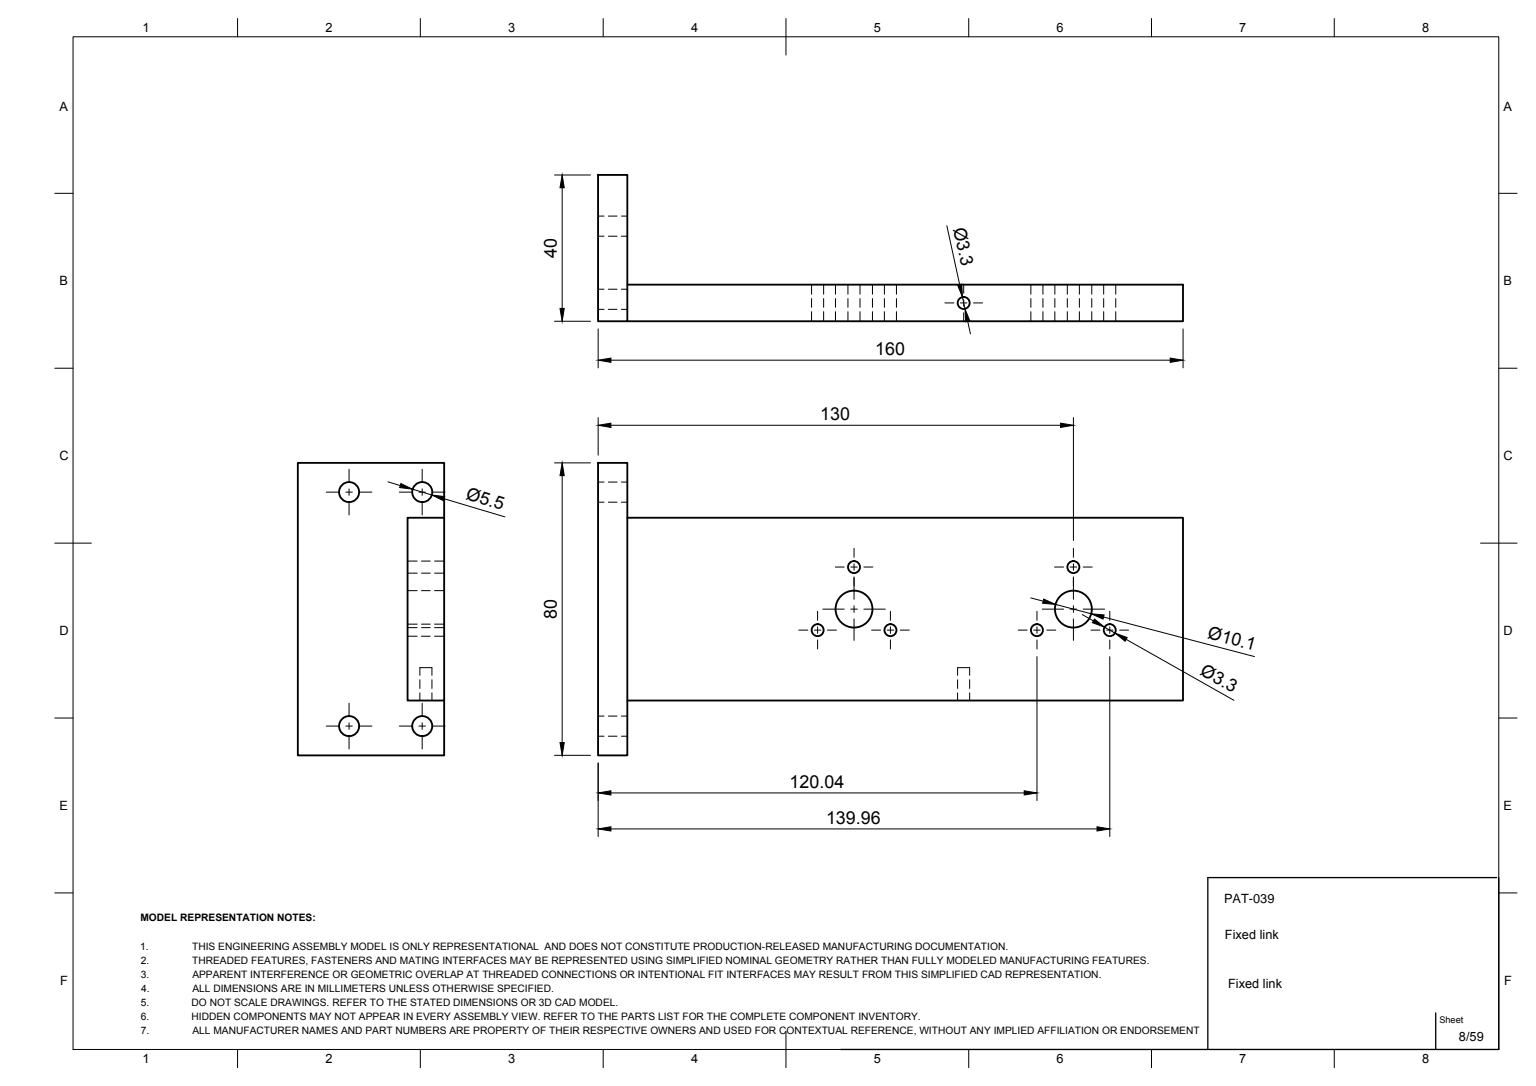
ISO-10303-21;
HEADER;
/* Generated by software containing ST-Developer
 * from STEP Tools, Inc. (www.steptools.com) 
 */

FILE_DESCRIPTION(
/* description */ ('Four-bar parallelogram arm'),
/* implementation_level */ '2;1');

FILE_NAME(
/* name */ 'Fixed link.step',
/* time_stamp */ '2026-10-28T03:24:55-07:00',
/* author */ (''),
/* organization */ (''),
/* preprocessor_version */ 'ST-DEVELOPER v20.2',
/* originating_system */ 'Autodesk Translation Framework v15.17.0.0',
/* authorisation */ '');

FILE_SCHEMA (('AUTOMOTIVE_DESIGN { 1 0 10303 214 3 1 1 }'));
ENDSEC;

DATA;
#10=MECHANICAL_DESIGN_GEOMETRIC_PRESENTATION_REPRESENTATION('',(#625),#14512);
#525=SHAPE_REPRESENTATION_RELATIONSHIP('SRR','None',#14746,#575);
#575=ADVANCED_BREP_SHAPE_REPRESENTATION('',(#683),#14461);
#625=STYLED_ITEM('',(#15101),#683);
#683=MANIFOLD_SOLID_BREP('Body1',#7329);
#743=FACE_BOUND('',#1666,.T.);
#744=FACE_BOUND('',#1667,.T.);
#745=FACE_BOUND('',#1668,.T.);
#746=FACE_BOUND('',#1669,.T.);
#747=FACE_BOUND('',#1672,.T.);
#748=FACE_BOUND('',#1673,.T.);
#749=FACE_BOUND('',#1674,.T.);
#750=FACE_BOUND('',#1675,.T.);
#751=FACE_BOUND('',#1679,.T.);
#752=FACE_BOUND('',#1680,.T.);
#753=FACE_BOUND('',#1681,.T.);
#754=FACE_BOUND('',#1682,.T.);
#755=FACE_BOUND('',#1683,.T.);
#756=FACE_BOUND('',#1684,.T.);
#757=FACE_BOUND('',#1685,.T.);
#758=FACE_BOUND('',#1686,.T.);
#759=FACE_BOUND('',#1689,.T.);
#760=FACE_BOUND('',#1690,.T.);
#761=FACE_BOUND('',#1691,.T.);
#762=FACE_BOUND('',#1692,.T.);
#763=FACE_BOUND('',#1693,.T.);
#764=FACE_BOUND('',#1694,.T.);
#765=FACE_BOUND('',#1695,.T.);
#766=FACE_BOUND('',#1696,.T.);
#767=FACE_BOUND('',#1698,.T.);
#1024=PLANE('',#7977);
#1025=PLANE('',#8014);
#1026=PLANE('',#8015);
#1027=PLANE('',#8016);
#1028=PLANE('',#8017);
#1029=PLANE('',#8018);
#1030=PLANE('',#8019);
#1031=PLANE('',#8020);
#1032=PLANE('',#8021);
#1033=PLANE('',#8022);
#1034=PLANE('',#8023);
#1223=FACE_OUTER_BOUND('',#1651,.T.);
#1224=FACE_OUTER_BOUND('',#1652,.T.);
#1225=FACE_OUTER_BOUND('',#1653,.T.);
#1226=FACE_OUTER_BOUND('',#1654,.T.);
#1227=FACE_OUTER_BOUND('',#1655,.T.);
#1228=FACE_OUTER_BOUND('',#1656,.T.);
#1229=FACE_OUTER_BOUND('',#1657,.T.);
#1230=FACE_OUTER_BOUND('',#1658,.T.);
#1231=FACE_OUTER_BOUND('',#1659,.T.);
#1232=FACE_OUTER_BOUND('',#1660,.T.);
#1233=FACE_OUTER_BOUND('',#1661,.T.);
#1234=FACE_OUTER_BOUND('',#1662,.T.);
#1235=FACE_OUTER_BOUND('',#1663,.T.);
#1236=FACE_OUTER_BOUND('',#1664,.T.);
#1237=FACE_OUTER_BOUND('',#1665,.T.);
#1238=FACE_OUTER_BOUND('',#1670,.T.);
#1239=FACE_OUTER_BOUND('',#1671,.T.);
#1240=FACE_OUTER_BOUND('',#1676,.T.);
#1241=FACE_OUTER_BOUND('',#1677,.T.);
#1242=FACE_OUTER_BOUND('',#1678,.T.);
#1243=FACE_OUTER_BOUND('',#1687,.T.);
#1244=FACE_OUTER_BOUND('',#1688,.T.);
#1245=FACE_OUTER_BOUND('',#1697,.T.);
#1246=FACE_OUTER_BOUND('',#1699,.T.);
#1651=EDGE_LOOP('',(#5084,#5085,#5086,#5087));
#1652=EDGE_LOOP('',(#5088));
#1653=EDGE_LOOP('',(#5089,#5090,#5091,#5092));
#1654=EDGE_LOOP('',(#5093,#5094,#5095,#5096));
#1655=EDGE_LOOP('',(#5097,#5098,#5099,#5100));
#1656=EDGE_LOOP('',(#5101,#5102,#5103,#5104));
#1657=EDGE_LOOP('',(#5105,#5106,#5107,#5108));
#1658=EDGE_LOOP('',(#5109,#5110,#5111,#5112));
#1659=EDGE_LOOP('',(#5113,#5114,#5115,#5116));
#1660=EDGE_LOOP('',(#5117,#5118,#5119,#5120));
#1661=EDGE_LOOP('',(#5121,#5122,#5123,#5124));
#1662=EDGE_LOOP('',(#5125,#5126,#5127,#5128));
#1663=EDGE_LOOP('',(#5129,#5130,#5131,#5132));
#1664=EDGE_LOOP('',(#5133,#5134,#5135,#5136));
#1665=EDGE_LOOP('',(#5137,#5138,#5139,#5140,#5141,#5142,#5143,#5144));
#1666=EDGE_LOOP('',(#5145));
#1667=EDGE_LOOP('',(#5146));
#1668=EDGE_LOOP('',(#5147));
#1669=EDGE_LOOP('',(#5148));
#1670=EDGE_LOOP('',(#5149,#5150,#5151,#5152));
#1671=EDGE_LOOP('',(#5153,#5154,#5155,#5156));
#1672=EDGE_LOOP('',(#5157));
#1673=EDGE_LOOP('',(#5158));
#1674=EDGE_LOOP('',(#5159));
#1675=EDGE_LOOP('',(#5160));
#1676=EDGE_LOOP('',(#5161,#5162,#5163,#5164));
#1677=EDGE_LOOP('',(#5165,#5166,#5167,#5168));
#1678=EDGE_LOOP('',(#5169,#5170,#5171,#5172));
#1679=EDGE_LOOP('',(#5173));
#1680=EDGE_LOOP('',(#5174));
#1681=EDGE_LOOP('',(#5175));
#1682=EDGE_LOOP('',(#5176));
#1683=EDGE_LOOP('',(#5177));
#1684=EDGE_LOOP('',(#5178));
#1685=EDGE_LOOP('',(#5179));
#1686=EDGE_LOOP('',(#5180));
#1687=EDGE_LOOP('',(#5181,#5182,#5183,#5184));
#1688=EDGE_LOOP('',(#5185,#5186,#5187,#5188,#5189,#5190,#5191,#5192));
#1689=EDGE_LOOP('',(#5193));
#1690=EDGE_LOOP('',(#5194));
#1691=EDGE_LOOP('',(#5195));
#1692=EDGE_LOOP('',(#5196));
#1693=EDGE_LOOP('',(#5197));
#1694=EDGE_LOOP('',(#5198));
#1695=EDGE_LOOP('',(#5199));
#1696=EDGE_LOOP('',(#5200));
#1697=EDGE_LOOP('',(#5201,#5202,#5203,#5204));
#1698=EDGE_LOOP('',(#5205));
#1699=EDGE_LOOP('',(#5206,#5207,#5208,#5209));
#2352=LINE('',#11540,#2746);
#2353=LINE('',#11547,#2747);
#2354=LINE('',#11553,#2748);
#2355=LINE('',#11559,#2749);
#2356=LINE('',#11565,#2750);
#2357=LINE('',#11571,#2751);
#2358=LINE('',#11577,#2752);
#2359=LINE('',#11583,#2753);
#2360=LINE('',#11589,#2754);
#2361=LINE('',#11595,#2755);
#2362=LINE('',#11601,#2756);
#2363=LINE('',#11607,#2757);
#2364=LINE('',#11613,#2758);
#2365=LINE('',#11618,#2759);
#2366=LINE('',#11620,#2760);
#2367=LINE('',#11622,#2761);
#2368=LINE('',#11624,#2762);
#2369=LINE('',#11626,#2763);
#2370=LINE('',#11628,#2764);
#2371=LINE('',#11630,#2765);
#2372=LINE('',#11631,#2766);
#2373=LINE('',#11634,#2767);
#2374=LINE('',#11636,#2768);
#2375=LINE('',#11637,#2769);
#2376=LINE('',#11640,#2770);
#2377=LINE('',#11642,#2771);
#2378=LINE('',#11643,#2772);
#2379=LINE('',#11645,#2773);
#2380=LINE('',#11646,#2774);
#2381=LINE('',#11650,#2775);
#2382=LINE('',#11652,#2776);
#2383=LINE('',#11653,#2777);
#2384=LINE('',#11656,#2778);
#2385=LINE('',#11657,#2779);
#2386=LINE('',#11660,#2780);
#2387=LINE('',#11661,#2781);
#2388=LINE('',#11663,#2782);
#2746=VECTOR('',#9086,0.164999999999999);
#2747=VECTOR('',#9095,0.165);
#2748=VECTOR('',#9102,0.165);
#2749=VECTOR('',#9109,0.165);
#2750=VECTOR('',#9116,0.505);
#2751=VECTOR('',#9123,0.165);
#2752=VECTOR('',#9130,0.165);
#2753=VECTOR('',#9137,0.165);
#2754=VECTOR('',#9144,0.505);
#2755=VECTOR('',#9151,0.275);
#2756=VECTOR('',#9158,0.275);
#2757=VECTOR('',#9165,0.275);
#2758=VECTOR('',#9172,0.275);
#2759=VECTOR('',#9177,1.);
#2760=VECTOR('',#9178,1.);
#2761=VECTOR('',#9179,1.);
#2762=VECTOR('',#9180,1.);
#2763=VECTOR('',#9181,1.);
#2764=VECTOR('',#9182,1.);
#2765=VECTOR('',#9183,1.);
#2766=VECTOR('',#9184,1.);
#2767=VECTOR('',#9187,1.);
#2768=VECTOR('',#9188,1.);
#2769=VECTOR('',#9189,1.);
#2770=VECTOR('',#9192,1.);
#2771=VECTOR('',#9193,1.);
#2772=VECTOR('',#9194,1.);
#2773=VECTOR('',#9197,1.);
#2774=VECTOR('',#9198,1.);
#2775=VECTOR('',#9203,1.);
#2776=VECTOR('',#9204,1.);
#2777=VECTOR('',#9205,1.);
#2778=VECTOR('',#9208,1.);
#2779=VECTOR('',#9209,1.);
#2780=VECTOR('',#9212,1.);
#2781=VECTOR('',#9213,1.);
#2782=VECTOR('',#9216,1.);
#3108=CIRCLE('',#7975,0.164999999999999);
#3109=CIRCLE('',#7976,0.164999999999999);
#3110=CIRCLE('',#7979,0.165);
#3111=CIRCLE('',#7980,0.165);
#3112=CIRCLE('',#7982,0.165);
#3113=CIRCLE('',#7983,0.165);
#3114=CIRCLE('',#7985,0.165);
#3115=CIRCLE('',#7986,0.165);
#3116=CIRCLE('',#7988,0.505);
#3117=CIRCLE('',#7989,0.505);
#3118=CIRCLE('',#7991,0.165);
#3119=CIRCLE('',#7992,0.165);
#3120=CIRCLE('',#7994,0.165);
#3121=CIRCLE('',#7995,0.165);
#3122=CIRCLE('',#7997,0.165);
#3123=CIRCLE('',#7998,0.165);
#3124=CIRCLE('',#8000,0.505);
#3125=CIRCLE('',#8001,0.505);
#3126=CIRCLE('',#8003,0.275);
#3127=CIRCLE('',#8004,0.275);
#3128=CIRCLE('',#8006,0.275);
#3129=CIRCLE('',#8007,0.275);
#3130=CIRCLE('',#8009,0.275);
#3131=CIRCLE('',#8010,0.275);
#3132=CIRCLE('',#8012,0.275);
#3133=CIRCLE('',#8013,0.275);
#3577=VERTEX_POINT('',#11537);
#3578=VERTEX_POINT('',#11539);
#3579=VERTEX_POINT('',#11544);
#3580=VERTEX_POINT('',#11546);
#3581=VERTEX_POINT('',#11550);
#3582=VERTEX_POINT('',#11552);
#3583=VERTEX_POINT('',#11556);
#3584=VERTEX_POINT('',#11558);
#3585=VERTEX_POINT('',#11562);
#3586=VERTEX_POINT('',#11564);
#3587=VERTEX_POINT('',#11568);
#3588=VERTEX_POINT('',#11570);
#3589=VERTEX_POINT('',#11574);
#3590=VERTEX_POINT('',#11576);
#3591=VERTEX_POINT('',#11580);
#3592=VERTEX_POINT('',#11582);
#3593=VERTEX_POINT('',#11586);
#3594=VERTEX_POINT('',#11588);
#3595=VERTEX_POINT('',#11592);
#3596=VERTEX_POINT('',#11594);
#3597=VERTEX_POINT('',#11598);
#3598=VERTEX_POINT('',#11600);
#3599=VERTEX_POINT('',#11604);
#3600=VERTEX_POINT('',#11606);
#3601=VERTEX_POINT('',#11610);
#3602=VERTEX_POINT('',#11612);
#3603=VERTEX_POINT('',#11616);
#3604=VERTEX_POINT('',#11617);
#3605=VERTEX_POINT('',#11619);
#3606=VERTEX_POINT('',#11621);
#3607=VERTEX_POINT('',#11623);
#3608=VERTEX_POINT('',#11625);
#3609=VERTEX_POINT('',#11627);
#3610=VERTEX_POINT('',#11629);
#3611=VERTEX_POINT('',#11633);
#3612=VERTEX_POINT('',#11635);
#3613=VERTEX_POINT('',#11639);
#3614=VERTEX_POINT('',#11641);
#3615=VERTEX_POINT('',#11649);
#3616=VERTEX_POINT('',#11651);
#3617=VERTEX_POINT('',#11655);
#3618=VERTEX_POINT('',#11659);
#4173=EDGE_CURVE('',#3577,#3577,#3108,.T.);
#4174=EDGE_CURVE('',#3577,#3578,#2352,.T.);
#4175=EDGE_CURVE('',#3578,#3578,#3109,.T.);
#4176=EDGE_CURVE('',#3579,#3579,#3110,.T.);
#4177=EDGE_CURVE('',#3579,#3580,#2353,.T.);
#4178=EDGE_CURVE('',#3580,#3580,#3111,.T.);
#4179=EDGE_CURVE('',#3581,#3581,#3112,.T.);
#4180=EDGE_CURVE('',#3581,#3582,#2354,.T.);
#4181=EDGE_CURVE('',#3582,#3582,#3113,.T.);
#4182=EDGE_CURVE('',#3583,#3583,#3114,.T.);
#4183=EDGE_CURVE('',#3583,#3584,#2355,.T.);
#4184=EDGE_CURVE('',#3584,#3584,#3115,.T.);
#4185=EDGE_CURVE('',#3585,#3585,#3116,.T.);
#4186=EDGE_CURVE('',#3585,#3586,#2356,.T.);
#4187=EDGE_CURVE('',#3586,#3586,#3117,.T.);
#4188=EDGE_CURVE('',#3587,#3587,#3118,.T.);
#4189=EDGE_CURVE('',#3587,#3588,#2357,.T.);
#4190=EDGE_CURVE('',#3588,#3588,#3119,.T.);
#4191=EDGE_CURVE('',#3589,#3589,#3120,.T.);
#4192=EDGE_CURVE('',#3589,#3590,#2358,.T.);
#4193=EDGE_CURVE('',#3590,#3590,#3121,.T.);
#4194=EDGE_CURVE('',#3591,#3591,#3122,.T.);
#4195=EDGE_CURVE('',#3591,#3592,#2359,.T.);
#4196=EDGE_CURVE('',#3592,#3592,#3123,.T.);
#4197=EDGE_CURVE('',#3593,#3593,#3124,.T.);
#4198=EDGE_CURVE('',#3593,#3594,#2360,.T.);
#4199=EDGE_CURVE('',#3594,#3594,#3125,.T.);
#4200=EDGE_CURVE('',#3595,#3595,#3126,.T.);
#4201=EDGE_CURVE('',#3595,#3596,#2361,.T.);
#4202=EDGE_CURVE('',#3596,#3596,#3127,.T.);
#4203=EDGE_CURVE('',#3597,#3597,#3128,.T.);
#4204=EDGE_CURVE('',#3597,#3598,#2362,.T.);
#4205=EDGE_CURVE('',#3598,#3598,#3129,.T.);
#4206=EDGE_CURVE('',#3599,#3599,#3130,.T.);
#4207=EDGE_CURVE('',#3599,#3600,#2363,.T.);
#4208=EDGE_CURVE('',#3600,#3600,#3131,.T.);
#4209=EDGE_CURVE('',#3601,#3601,#3132,.T.);
#4210=EDGE_CURVE('',#3601,#3602,#2364,.T.);
#4211=EDGE_CURVE('',#3602,#3602,#3133,.T.);
#4212=EDGE_CURVE('',#3603,#3604,#2365,.T.);
#4213=EDGE_CURVE('',#3605,#3603,#2366,.T.);
#4214=EDGE_CURVE('',#3606,#3605,#2367,.T.);
#4215=EDGE_CURVE('',#3607,#3606,#2368,.T.);
#4216=EDGE_CURVE('',#3607,#3608,#2369,.T.);
#4217=EDGE_CURVE('',#3609,#3608,#2370,.T.);
#4218=EDGE_CURVE('',#3610,#3609,#2371,.T.);
#4219=EDGE_CURVE('',#3604,#3610,#2372,.T.);
#4220=EDGE_CURVE('',#3610,#3611,#2373,.T.);
#4221=EDGE_CURVE('',#3612,#3609,#2374,.T.);
#4222=EDGE_CURVE('',#3611,#3612,#2375,.T.);
#4223=EDGE_CURVE('',#3611,#3613,#2376,.T.);
#4224=EDGE_CURVE('',#3614,#3612,#2377,.T.);
#4225=EDGE_CURVE('',#3613,#3614,#2378,.T.);
#4226=EDGE_CURVE('',#3613,#3607,#2379,.T.);
#4227=EDGE_CURVE('',#3608,#3614,#2380,.T.);
#4228=EDGE_CURVE('',#3603,#3615,#2381,.T.);
#4229=EDGE_CURVE('',#3616,#3615,#2382,.T.);
#4230=EDGE_CURVE('',#3605,#3616,#2383,.T.);
#4231=EDGE_CURVE('',#3617,#3616,#2384,.T.);
#4232=EDGE_CURVE('',#3606,#3617,#2385,.T.);
#4233=EDGE_CURVE('',#3618,#3617,#2386,.T.);
#4234=EDGE_CURVE('',#3604,#3618,#2387,.T.);
#4235=EDGE_CURVE('',#3615,#3618,#2388,.T.);
#5084=ORIENTED_EDGE('',*,*,#4173,.F.);
#5085=ORIENTED_EDGE('',*,*,#4174,.T.);
#5086=ORIENTED_EDGE('',*,*,#4175,.T.);
#5087=ORIENTED_EDGE('',*,*,#4174,.F.);
#5088=ORIENTED_EDGE('',*,*,#4175,.F.);
#5089=ORIENTED_EDGE('',*,*,#4176,.F.);
#5090=ORIENTED_EDGE('',*,*,#4177,.T.);
#5091=ORIENTED_EDGE('',*,*,#4178,.F.);
#5092=ORIENTED_EDGE('',*,*,#4177,.F.);
#5093=ORIENTED_EDGE('',*,*,#4179,.F.);
#5094=ORIENTED_EDGE('',*,*,#4180,.T.);
#5095=ORIENTED_EDGE('',*,*,#4181,.F.);
#5096=ORIENTED_EDGE('',*,*,#4180,.F.);
#5097=ORIENTED_EDGE('',*,*,#4182,.F.);
#5098=ORIENTED_EDGE('',*,*,#4183,.T.);
#5099=ORIENTED_EDGE('',*,*,#4184,.F.);
#5100=ORIENTED_EDGE('',*,*,#4183,.F.);
#5101=ORIENTED_EDGE('',*,*,#4185,.F.);
#5102=ORIENTED_EDGE('',*,*,#4186,.T.);
#5103=ORIENTED_EDGE('',*,*,#4187,.F.);
#5104=ORIENTED_EDGE('',*,*,#4186,.F.);
#5105=ORIENTED_EDGE('',*,*,#4188,.F.);
#5106=ORIENTED_EDGE('',*,*,#4189,.T.);
#5107=ORIENTED_EDGE('',*,*,#4190,.F.);
#5108=ORIENTED_EDGE('',*,*,#4189,.F.);
#5109=ORIENTED_EDGE('',*,*,#4191,.F.);
#5110=ORIENTED_EDGE('',*,*,#4192,.T.);
#5111=ORIENTED_EDGE('',*,*,#4193,.F.);
#5112=ORIENTED_EDGE('',*,*,#4192,.F.);
#5113=ORIENTED_EDGE('',*,*,#4194,.F.);
#5114=ORIENTED_EDGE('',*,*,#4195,.T.);
#5115=ORIENTED_EDGE('',*,*,#4196,.F.);
#5116=ORIENTED_EDGE('',*,*,#4195,.F.);
#5117=ORIENTED_EDGE('',*,*,#4197,.F.);
#5118=ORIENTED_EDGE('',*,*,#4198,.T.);
#5119=ORIENTED_EDGE('',*,*,#4199,.F.);
#5120=ORIENTED_EDGE('',*,*,#4198,.F.);
#5121=ORIENTED_EDGE('',*,*,#4200,.F.);
#5122=ORIENTED_EDGE('',*,*,#4201,.T.);
#5123=ORIENTED_EDGE('',*,*,#4202,.F.);
#5124=ORIENTED_EDGE('',*,*,#4201,.F.);
#5125=ORIENTED_EDGE('',*,*,#4203,.F.);
#5126=ORIENTED_EDGE('',*,*,#4204,.T.);
#5127=ORIENTED_EDGE('',*,*,#4205,.F.);
#5128=ORIENTED_EDGE('',*,*,#4204,.F.);
#5129=ORIENTED_EDGE('',*,*,#4206,.F.);
#5130=ORIENTED_EDGE('',*,*,#4207,.T.);
#5131=ORIENTED_EDGE('',*,*,#4208,.F.);
#5132=ORIENTED_EDGE('',*,*,#4207,.F.);
#5133=ORIENTED_EDGE('',*,*,#4209,.F.);
#5134=ORIENTED_EDGE('',*,*,#4210,.T.);
#5135=ORIENTED_EDGE('',*,*,#4211,.F.);
#5136=ORIENTED_EDGE('',*,*,#4210,.F.);
#5137=ORIENTED_EDGE('',*,*,#4212,.F.);
#5138=ORIENTED_EDGE('',*,*,#4213,.F.);
#5139=ORIENTED_EDGE('',*,*,#4214,.F.);
#5140=ORIENTED_EDGE('',*,*,#4215,.F.);
#5141=ORIENTED_EDGE('',*,*,#4216,.T.);
#5142=ORIENTED_EDGE('',*,*,#4217,.F.);
#5143=ORIENTED_EDGE('',*,*,#4218,.F.);
#5144=ORIENTED_EDGE('',*,*,#4219,.F.);
#5145=ORIENTED_EDGE('',*,*,#4202,.T.);
#5146=ORIENTED_EDGE('',*,*,#4205,.T.);
#5147=ORIENTED_EDGE('',*,*,#4208,.T.);
#5148=ORIENTED_EDGE('',*,*,#4211,.T.);
#5149=ORIENTED_EDGE('',*,*,#4220,.F.);
#5150=ORIENTED_EDGE('',*,*,#4218,.T.);
#5151=ORIENTED_EDGE('',*,*,#4221,.F.);
#5152=ORIENTED_EDGE('',*,*,#4222,.F.);
#5153=ORIENTED_EDGE('',*,*,#4223,.F.);
#5154=ORIENTED_EDGE('',*,*,#4222,.T.);
#5155=ORIENTED_EDGE('',*,*,#4224,.F.);
#5156=ORIENTED_EDGE('',*,*,#4225,.F.);
#5157=ORIENTED_EDGE('',*,*,#4200,.T.);
#5158=ORIENTED_EDGE('',*,*,#4203,.T.);
#5159=ORIENTED_EDGE('',*,*,#4206,.T.);
#5160=ORIENTED_EDGE('',*,*,#4209,.T.);
#5161=ORIENTED_EDGE('',*,*,#4226,.F.);
#5162=ORIENTED_EDGE('',*,*,#4225,.T.);
#5163=ORIENTED_EDGE('',*,*,#4227,.F.);
#5164=ORIENTED_EDGE('',*,*,#4216,.F.);
#5165=ORIENTED_EDGE('',*,*,#4217,.T.);
#5166=ORIENTED_EDGE('',*,*,#4227,.T.);
#5167=ORIENTED_EDGE('',*,*,#4224,.T.);
#5168=ORIENTED_EDGE('',*,*,#4221,.T.);
#5169=ORIENTED_EDGE('',*,*,#4213,.T.);
#5170=ORIENTED_EDGE('',*,*,#4228,.T.);
#5171=ORIENTED_EDGE('',*,*,#4229,.F.);
#5172=ORIENTED_EDGE('',*,*,#4230,.F.);
#5173=ORIENTED_EDGE('',*,*,#4199,.T.);
#5174=ORIENTED_EDGE('',*,*,#4196,.T.);
#5175=ORIENTED_EDGE('',*,*,#4193,.T.);
#5176=ORIENTED_EDGE('',*,*,#4190,.T.);
#5177=ORIENTED_EDGE('',*,*,#4187,.T.);
#5178=ORIENTED_EDGE('',*,*,#4184,.T.);
#5179=ORIENTED_EDGE('',*,*,#4181,.T.);
#5180=ORIENTED_EDGE('',*,*,#4178,.T.);
#5181=ORIENTED_EDGE('',*,*,#4214,.T.);
#5182=ORIENTED_EDGE('',*,*,#4230,.T.);
#5183=ORIENTED_EDGE('',*,*,#4231,.F.);
#5184=ORIENTED_EDGE('',*,*,#4232,.F.);
#5185=ORIENTED_EDGE('',*,*,#4232,.T.);
#5186=ORIENTED_EDGE('',*,*,#4233,.F.);
#5187=ORIENTED_EDGE('',*,*,#4234,.F.);
#5188=ORIENTED_EDGE('',*,*,#4219,.T.);
#5189=ORIENTED_EDGE('',*,*,#4220,.T.);
#5190=ORIENTED_EDGE('',*,*,#4223,.T.);
#5191=ORIENTED_EDGE('',*,*,#4226,.T.);
#5192=ORIENTED_EDGE('',*,*,#4215,.T.);
#5193=ORIENTED_EDGE('',*,*,#4197,.T.);
#5194=ORIENTED_EDGE('',*,*,#4194,.T.);
#5195=ORIENTED_EDGE('',*,*,#4191,.T.);
#5196=ORIENTED_EDGE('',*,*,#4188,.T.);
#5197=ORIENTED_EDGE('',*,*,#4185,.T.);
#5198=ORIENTED_EDGE('',*,*,#4182,.T.);
#5199=ORIENTED_EDGE('',*,*,#4179,.T.);
#5200=ORIENTED_EDGE('',*,*,#4176,.T.);
#5201=ORIENTED_EDGE('',*,*,#4212,.T.);
#5202=ORIENTED_EDGE('',*,*,#4234,.T.);
#5203=ORIENTED_EDGE('',*,*,#4235,.F.);
#5204=ORIENTED_EDGE('',*,*,#4228,.F.);
#5205=ORIENTED_EDGE('',*,*,#4173,.T.);
#5206=ORIENTED_EDGE('',*,*,#4235,.T.);
#5207=ORIENTED_EDGE('',*,*,#4233,.T.);
#5208=ORIENTED_EDGE('',*,*,#4231,.T.);
#5209=ORIENTED_EDGE('',*,*,#4229,.T.);
#6718=CYLINDRICAL_SURFACE('',#7974,0.164999999999999);
#6719=CYLINDRICAL_SURFACE('',#7978,0.165);
#6720=CYLINDRICAL_SURFACE('',#7981,0.165);
#6721=CYLINDRICAL_SURFACE('',#7984,0.165);
#6722=CYLINDRICAL_SURFACE('',#7987,0.505);
#6723=CYLINDRICAL_SURFACE('',#7990,0.165);
#6724=CYLINDRICAL_SURFACE('',#7993,0.165);
#6725=CYLINDRICAL_SURFACE('',#7996,0.165);
#6726=CYLINDRICAL_SURFACE('',#7999,0.505);
#6727=CYLINDRICAL_SURFACE('',#8002,0.275);
#6728=CYLINDRICAL_SURFACE('',#8005,0.275);
#6729=CYLINDRICAL_SURFACE('',#8008,0.275);
#6730=CYLINDRICAL_SURFACE('',#8011,0.275);
#6928=ADVANCED_FACE('',(#1223),#6718,.F.);
#6929=ADVANCED_FACE('',(#1224),#1024,.F.);
#6930=ADVANCED_FACE('',(#1225),#6719,.F.);
#6931=ADVANCED_FACE('',(#1226),#6720,.F.);
#6932=ADVANCED_FACE('',(#1227),#6721,.F.);
#6933=ADVANCED_FACE('',(#1228),#6722,.F.);
#6934=ADVANCED_FACE('',(#1229),#6723,.F.);
#6935=ADVANCED_FACE('',(#1230),#6724,.F.);
#6936=ADVANCED_FACE('',(#1231),#6725,.F.);
#6937=ADVANCED_FACE('',(#1232),#6726,.F.);
#6938=ADVANCED_FACE('',(#1233),#6727,.F.);
#6939=ADVANCED_FACE('',(#1234),#6728,.F.);
#6940=ADVANCED_FACE('',(#1235),#6729,.F.);
#6941=ADVANCED_FACE('',(#1236),#6730,.F.);
#6942=ADVANCED_FACE('',(#1237,#743,#744,#745,#746),#1025,.T.);
#6943=ADVANCED_FACE('',(#1238),#1026,.T.);
#6944=ADVANCED_FACE('',(#1239,#747,#748,#749,#750),#1027,.T.);
#6945=ADVANCED_FACE('',(#1240),#1028,.T.);
#6946=ADVANCED_FACE('',(#1241),#1029,.T.);
#6947=ADVANCED_FACE('',(#1242,#751,#752,#753,#754,#755,#756,#757,#758),
#1030,.T.);
#6948=ADVANCED_FACE('',(#1243),#1031,.T.);
#6949=ADVANCED_FACE('',(#1244,#759,#760,#761,#762,#763,#764,#765,#766),
#1032,.T.);
#6950=ADVANCED_FACE('',(#1245,#767),#1033,.T.);
#6951=ADVANCED_FACE('',(#1246),#1034,.T.);
#7329=CLOSED_SHELL('',(#6928,#6929,#6930,#6931,#6932,#6933,#6934,#6935,
#6936,#6937,#6938,#6939,#6940,#6941,#6942,#6943,#6944,#6945,#6946,#6947,
#6948,#6949,#6950,#6951));
#7973=AXIS2_PLACEMENT_3D('',#11535,#9080,#9081);
#7974=AXIS2_PLACEMENT_3D('',#11536,#9082,#9083);
#7975=AXIS2_PLACEMENT_3D('',#11538,#9084,#9085);
#7976=AXIS2_PLACEMENT_3D('',#11541,#9087,#9088);
#7977=AXIS2_PLACEMENT_3D('',#11542,#9089,#9090);
#7978=AXIS2_PLACEMENT_3D('',#11543,#9091,#9092);
#7979=AXIS2_PLACEMENT_3D('',#11545,#9093,#9094);
#7980=AXIS2_PLACEMENT_3D('',#11548,#9096,#9097);
#7981=AXIS2_PLACEMENT_3D('',#11549,#9098,#9099);
#7982=AXIS2_PLACEMENT_3D('',#11551,#9100,#9101);
#7983=AXIS2_PLACEMENT_3D('',#11554,#9103,#9104);
#7984=AXIS2_PLACEMENT_3D('',#11555,#9105,#9106);
#7985=AXIS2_PLACEMENT_3D('',#11557,#9107,#9108);
#7986=AXIS2_PLACEMENT_3D('',#11560,#9110,#9111);
#7987=AXIS2_PLACEMENT_3D('',#11561,#9112,#9113);
#7988=AXIS2_PLACEMENT_3D('',#11563,#9114,#9115);
#7989=AXIS2_PLACEMENT_3D('',#11566,#9117,#9118);
#7990=AXIS2_PLACEMENT_3D('',#11567,#9119,#9120);
#7991=AXIS2_PLACEMENT_3D('',#11569,#9121,#9122);
#7992=AXIS2_PLACEMENT_3D('',#11572,#9124,#9125);
#7993=AXIS2_PLACEMENT_3D('',#11573,#9126,#9127);
#7994=AXIS2_PLACEMENT_3D('',#11575,#9128,#9129);
#7995=AXIS2_PLACEMENT_3D('',#11578,#9131,#9132);
#7996=AXIS2_PLACEMENT_3D('',#11579,#9133,#9134);
#7997=AXIS2_PLACEMENT_3D('',#11581,#9135,#9136);
#7998=AXIS2_PLACEMENT_3D('',#11584,#9138,#9139);
#7999=AXIS2_PLACEMENT_3D('',#11585,#9140,#9141);
#8000=AXIS2_PLACEMENT_3D('',#11587,#9142,#9143);
#8001=AXIS2_PLACEMENT_3D('',#11590,#9145,#9146);
#8002=AXIS2_PLACEMENT_3D('',#11591,#9147,#9148);
#8003=AXIS2_PLACEMENT_3D('',#11593,#9149,#9150);
#8004=AXIS2_PLACEMENT_3D('',#11596,#9152,#9153);
#8005=AXIS2_PLACEMENT_3D('',#11597,#9154,#9155);
#8006=AXIS2_PLACEMENT_3D('',#11599,#9156,#9157);
#8007=AXIS2_PLACEMENT_3D('',#11602,#9159,#9160);
#8008=AXIS2_PLACEMENT_3D('',#11603,#9161,#9162);
#8009=AXIS2_PLACEMENT_3D('',#11605,#9163,#9164);
#8010=AXIS2_PLACEMENT_3D('',#11608,#9166,#9167);
#8011=AXIS2_PLACEMENT_3D('',#11609,#9168,#9169);
#8012=AXIS2_PLACEMENT_3D('',#11611,#9170,#9171);
#8013=AXIS2_PLACEMENT_3D('',#11614,#9173,#9174);
#8014=AXIS2_PLACEMENT_3D('',#11615,#9175,#9176);
#8015=AXIS2_PLACEMENT_3D('',#11632,#9185,#9186);
#8016=AXIS2_PLACEMENT_3D('',#11638,#9190,#9191);
#8017=AXIS2_PLACEMENT_3D('',#11644,#9195,#9196);
#8018=AXIS2_PLACEMENT_3D('',#11647,#9199,#9200);
#8019=AXIS2_PLACEMENT_3D('',#11648,#9201,#9202);
#8020=AXIS2_PLACEMENT_3D('',#11654,#9206,#9207);
#8021=AXIS2_PLACEMENT_3D('',#11658,#9210,#9211);
#8022=AXIS2_PLACEMENT_3D('',#11662,#9214,#9215);
#8023=AXIS2_PLACEMENT_3D('',#11664,#9217,#9218);
#9080=DIRECTION('axis',(0.,0.,1.));
#9081=DIRECTION('refdir',(1.,0.,0.));
#9082=DIRECTION('center_axis',(1.,0.,0.));
#9083=DIRECTION('ref_axis',(0.,0.,-1.));
#9084=DIRECTION('center_axis',(1.,0.,0.));
#9085=DIRECTION('ref_axis',(0.,0.,-1.));
#9086=DIRECTION('',(1.,0.,0.));
#9087=DIRECTION('center_axis',(1.,0.,0.));
#9088=DIRECTION('ref_axis',(0.,0.,-1.));
#9089=DIRECTION('center_axis',(1.,0.,0.));
#9090=DIRECTION('ref_axis',(0.,0.,-1.));
#9091=DIRECTION('center_axis',(0.,1.,0.));
#9092=DIRECTION('ref_axis',(1.,0.,0.));
#9093=DIRECTION('center_axis',(0.,1.,0.));
#9094=DIRECTION('ref_axis',(1.,0.,0.));
#9095=DIRECTION('',(0.,1.,0.));
#9096=DIRECTION('center_axis',(0.,-1.,0.));
#9097=DIRECTION('ref_axis',(1.,0.,0.));
#9098=DIRECTION('center_axis',(0.,1.,0.));
#9099=DIRECTION('ref_axis',(1.,0.,0.));
#9100=DIRECTION('center_axis',(0.,1.,0.));
#9101=DIRECTION('ref_axis',(1.,0.,0.));
#9102=DIRECTION('',(0.,1.,0.));
#9103=DIRECTION('center_axis',(0.,-1.,0.));
#9104=DIRECTION('ref_axis',(1.,0.,0.));
#9105=DIRECTION('center_axis',(0.,1.,0.));
#9106=DIRECTION('ref_axis',(1.,0.,0.));
#9107=DIRECTION('center_axis',(0.,1.,0.));
#9108=DIRECTION('ref_axis',(1.,0.,0.));
#9109=DIRECTION('',(0.,1.,0.));
#9110=DIRECTION('center_axis',(0.,-1.,0.));
#9111=DIRECTION('ref_axis',(1.,0.,0.));
#9112=DIRECTION('center_axis',(0.,1.,0.));
#9113=DIRECTION('ref_axis',(1.,0.,0.));
#9114=DIRECTION('center_axis',(0.,1.,0.));
#9115=DIRECTION('ref_axis',(1.,0.,0.));
#9116=DIRECTION('',(0.,1.,0.));
#9117=DIRECTION('center_axis',(0.,-1.,0.));
#9118=DIRECTION('ref_axis',(1.,0.,0.));
#9119=DIRECTION('center_axis',(0.,1.,0.));
#9120=DIRECTION('ref_axis',(1.,0.,0.));
#9121=DIRECTION('center_axis',(0.,1.,0.));
#9122=DIRECTION('ref_axis',(1.,0.,0.));
#9123=DIRECTION('',(0.,1.,0.));
#9124=DIRECTION('center_axis',(0.,-1.,0.));
#9125=DIRECTION('ref_axis',(1.,0.,0.));
#9126=DIRECTION('center_axis',(0.,1.,0.));
#9127=DIRECTION('ref_axis',(1.,0.,0.));
#9128=DIRECTION('center_axis',(0.,1.,0.));
#9129=DIRECTION('ref_axis',(1.,0.,0.));
#9130=DIRECTION('',(0.,1.,0.));
#9131=DIRECTION('center_axis',(0.,-1.,0.));
#9132=DIRECTION('ref_axis',(1.,0.,0.));
#9133=DIRECTION('center_axis',(0.,1.,0.));
#9134=DIRECTION('ref_axis',(1.,0.,0.));
#9135=DIRECTION('center_axis',(0.,1.,0.));
#9136=DIRECTION('ref_axis',(1.,0.,0.));
#9137=DIRECTION('',(0.,1.,0.));
#9138=DIRECTION('center_axis',(0.,-1.,0.));
#9139=DIRECTION('ref_axis',(1.,0.,0.));
#9140=DIRECTION('center_axis',(0.,1.,0.));
#9141=DIRECTION('ref_axis',(1.,0.,0.));
#9142=DIRECTION('center_axis',(0.,1.,0.));
#9143=DIRECTION('ref_axis',(1.,0.,0.));
#9144=DIRECTION('',(0.,1.,0.));
#9145=DIRECTION('center_axis',(0.,-1.,0.));
#9146=DIRECTION('ref_axis',(1.,0.,0.));
#9147=DIRECTION('center_axis',(0.,0.,1.));
#9148=DIRECTION('ref_axis',(1.,0.,0.));
#9149=DIRECTION('center_axis',(0.,0.,1.));
#9150=DIRECTION('ref_axis',(1.,0.,0.));
#9151=DIRECTION('',(0.,0.,1.));
#9152=DIRECTION('center_axis',(0.,0.,-1.));
#9153=DIRECTION('ref_axis',(1.,0.,0.));
#9154=DIRECTION('center_axis',(0.,0.,1.));
#9155=DIRECTION('ref_axis',(1.,0.,0.));
#9156=DIRECTION('center_axis',(0.,0.,1.));
#9157=DIRECTION('ref_axis',(1.,0.,0.));
#9158=DIRECTION('',(0.,0.,1.));
#9159=DIRECTION('center_axis',(0.,0.,-1.));
#9160=DIRECTION('ref_axis',(1.,0.,0.));
#9161=DIRECTION('center_axis',(0.,0.,1.));
#9162=DIRECTION('ref_axis',(1.,0.,0.));
#9163=DIRECTION('center_axis',(0.,0.,1.));
#9164=DIRECTION('ref_axis',(1.,0.,0.));
#9165=DIRECTION('',(0.,0.,1.));
#9166=DIRECTION('center_axis',(0.,0.,-1.));
#9167=DIRECTION('ref_axis',(1.,0.,0.));
#9168=DIRECTION('center_axis',(0.,0.,1.));
#9169=DIRECTION('ref_axis',(1.,0.,0.));
#9170=DIRECTION('center_axis',(0.,0.,1.));
#9171=DIRECTION('ref_axis',(1.,0.,0.));
#9172=DIRECTION('',(0.,0.,1.));
#9173=DIRECTION('center_axis',(0.,0.,-1.));
#9174=DIRECTION('ref_axis',(1.,0.,0.));
#9175=DIRECTION('center_axis',(0.,0.,1.));
#9176=DIRECTION('ref_axis',(1.,0.,0.));
#9177=DIRECTION('',(0.,-1.,0.));
#9178=DIRECTION('',(-1.,0.,0.));
#9179=DIRECTION('',(0.,1.,0.));
#9180=DIRECTION('',(-1.,0.,0.));
#9181=DIRECTION('',(0.,1.,0.));
#9182=DIRECTION('',(1.,0.,0.));
#9183=DIRECTION('',(0.,1.,0.));
#9184=DIRECTION('',(-1.,0.,0.));
#9185=DIRECTION('center_axis',(-1.,0.,0.));
#9186=DIRECTION('ref_axis',(0.,0.,1.));
#9187=DIRECTION('',(0.,0.,-1.));
#9188=DIRECTION('',(0.,0.,1.));
#9189=DIRECTION('',(0.,1.,0.));
#9190=DIRECTION('center_axis',(0.,0.,-1.));
#9191=DIRECTION('ref_axis',(-1.,0.,0.));
#9192=DIRECTION('',(1.,0.,0.));
#9193=DIRECTION('',(-1.,0.,0.));
#9194=DIRECTION('',(0.,1.,0.));
#9195=DIRECTION('center_axis',(1.,0.,0.));
#9196=DIRECTION('ref_axis',(0.,0.,-1.));
#9197=DIRECTION('',(0.,0.,1.));
#9198=DIRECTION('',(0.,0.,-1.));
#9199=DIRECTION('center_axis',(0.,1.,0.));
#9200=DIRECTION('ref_axis',(0.,0.,1.));
#9201=DIRECTION('center_axis',(0.,1.,0.));
#9202=DIRECTION('ref_axis',(-1.,0.,0.));
#9203=DIRECTION('',(0.,0.,1.));
#9204=DIRECTION('',(-1.,0.,0.));
#9205=DIRECTION('',(0.,0.,1.));
#9206=DIRECTION('center_axis',(1.,0.,0.));
#9207=DIRECTION('ref_axis',(0.,1.,0.));
#9208=DIRECTION('',(0.,1.,0.));
#9209=DIRECTION('',(0.,0.,1.));
#9210=DIRECTION('center_axis',(0.,-1.,0.));
#9211=DIRECTION('ref_axis',(1.,0.,0.));
#9212=DIRECTION('',(1.,0.,0.));
#9213=DIRECTION('',(0.,0.,1.));
#9214=DIRECTION('center_axis',(-1.,0.,0.));
#9215=DIRECTION('ref_axis',(0.,-1.,0.));
#9216=DIRECTION('',(0.,-1.,0.));
#9217=DIRECTION('center_axis',(0.,0.,1.));
#9218=DIRECTION('ref_axis',(1.,0.,0.));
#11535=CARTESIAN_POINT('',(0.,0.,0.));
#11536=CARTESIAN_POINT('Origin',(-2.6,3.4,11.));
#11537=CARTESIAN_POINT('',(-2.5,3.4,11.165));
#11538=CARTESIAN_POINT('Origin',(-2.5,3.4,11.));
#11539=CARTESIAN_POINT('',(-1.6,3.4,11.165));
#11540=CARTESIAN_POINT('',(-2.6,3.4,11.165));
#11541=CARTESIAN_POINT('Origin',(-1.6,3.4,11.));
#11542=CARTESIAN_POINT('Origin',(-1.6,3.4,11.));
#11543=CARTESIAN_POINT('Origin',(1.15,2.8,14.));
#11544=CARTESIAN_POINT('',(0.985,2.9,14.));
#11545=CARTESIAN_POINT('Origin',(1.15,2.9,14.));
#11546=CARTESIAN_POINT('',(0.985,3.9,14.));
#11547=CARTESIAN_POINT('',(0.985,2.8,14.));
#11548=CARTESIAN_POINT('Origin',(1.15,3.9,14.));
#11549=CARTESIAN_POINT('Origin',(-0.575,2.8,14.9959292143521));
#11550=CARTESIAN_POINT('',(-0.74,2.9,14.9959292143521));
#11551=CARTESIAN_POINT('Origin',(-0.575,2.9,14.9959292143521));
#11552=CARTESIAN_POINT('',(-0.74,3.9,14.9959292143521));
#11553=CARTESIAN_POINT('',(-0.74,2.8,14.9959292143521));
#11554=CARTESIAN_POINT('Origin',(-0.575,3.9,14.9959292143521));
#11555=CARTESIAN_POINT('Origin',(-0.575000000000001,2.8,13.0040707856479));
#11556=CARTESIAN_POINT('',(-0.74,2.9,13.0040707856479));
#11557=CARTESIAN_POINT('Origin',(-0.575000000000001,2.9,13.0040707856479));
#11558=CARTESIAN_POINT('',(-0.74,3.9,13.0040707856479));
#11559=CARTESIAN_POINT('',(-0.74,2.8,13.0040707856479));
#11560=CARTESIAN_POINT('Origin',(-0.575000000000001,3.9,13.0040707856479));
#11561=CARTESIAN_POINT('Origin',(0.,2.8,14.));
#11562=CARTESIAN_POINT('',(-0.505,2.9,14.));
#11563=CARTESIAN_POINT('Origin',(0.,2.9,14.));
#11564=CARTESIAN_POINT('',(-0.505,3.9,14.));
#11565=CARTESIAN_POINT('',(-0.505,2.8,14.));
#11566=CARTESIAN_POINT('Origin',(0.,3.9,14.));
#11567=CARTESIAN_POINT('Origin',(1.15,2.8,8.));
#11568=CARTESIAN_POINT('',(0.985,2.9,8.));
#11569=CARTESIAN_POINT('Origin',(1.15,2.9,8.));
#11570=CARTESIAN_POINT('',(0.985,3.9,8.));
#11571=CARTESIAN_POINT('',(0.985,2.8,8.));
#11572=CARTESIAN_POINT('Origin',(1.15,3.9,8.));
#11573=CARTESIAN_POINT('Origin',(-0.575,2.8,8.9959292143521));
#11574=CARTESIAN_POINT('',(-0.74,2.9,8.9959292143521));
#11575=CARTESIAN_POINT('Origin',(-0.575,2.9,8.9959292143521));
#11576=CARTESIAN_POINT('',(-0.74,3.9,8.9959292143521));
#11577=CARTESIAN_POINT('',(-0.74,2.8,8.9959292143521));
#11578=CARTESIAN_POINT('Origin',(-0.575,3.9,8.9959292143521));
#11579=CARTESIAN_POINT('Origin',(-0.575000000000001,2.8,7.0040707856479));
#11580=CARTESIAN_POINT('',(-0.74,2.9,7.0040707856479));
#11581=CARTESIAN_POINT('Origin',(-0.575000000000001,2.9,7.0040707856479));
#11582=CARTESIAN_POINT('',(-0.74,3.9,7.0040707856479));
#11583=CARTESIAN_POINT('',(-0.74,2.8,7.0040707856479));
#11584=CARTESIAN_POINT('Origin',(-0.575000000000001,3.9,7.0040707856479));
#11585=CARTESIAN_POINT('Origin',(0.,2.8,8.));
#11586=CARTESIAN_POINT('',(-0.505,2.9,8.));
#11587=CARTESIAN_POINT('Origin',(0.,2.9,8.));
#11588=CARTESIAN_POINT('',(-0.505,3.9,8.));
#11589=CARTESIAN_POINT('',(-0.505,2.8,8.));
#11590=CARTESIAN_POINT('Origin',(0.,3.9,8.));
#11591=CARTESIAN_POINT('Origin',(3.2,3.5,0.9));
#11592=CARTESIAN_POINT('',(2.925,3.5,1.));
#11593=CARTESIAN_POINT('Origin',(3.2,3.5,1.));
#11594=CARTESIAN_POINT('',(2.925,3.5,1.8));
#11595=CARTESIAN_POINT('',(2.925,3.5,0.9));
#11596=CARTESIAN_POINT('Origin',(3.2,3.5,1.8));
#11597=CARTESIAN_POINT('Origin',(-3.2,5.5,0.9));
#11598=CARTESIAN_POINT('',(-3.475,5.5,1.));
#11599=CARTESIAN_POINT('Origin',(-3.2,5.5,1.));
#11600=CARTESIAN_POINT('',(-3.475,5.5,1.8));
#11601=CARTESIAN_POINT('',(-3.475,5.5,0.9));
#11602=CARTESIAN_POINT('Origin',(-3.2,5.5,1.8));
#11603=CARTESIAN_POINT('Origin',(-3.2,3.5,0.9));
#11604=CARTESIAN_POINT('',(-3.475,3.5,1.));
#11605=CARTESIAN_POINT('Origin',(-3.2,3.5,1.));
#11606=CARTESIAN_POINT('',(-3.475,3.5,1.8));
#11607=CARTESIAN_POINT('',(-3.475,3.5,0.9));
#11608=CARTESIAN_POINT('Origin',(-3.2,3.5,1.8));
#11609=CARTESIAN_POINT('Origin',(3.2,5.5,0.9));
#11610=CARTESIAN_POINT('',(2.925,5.5,1.));
#11611=CARTESIAN_POINT('Origin',(3.2,5.5,1.));
#11612=CARTESIAN_POINT('',(2.925,5.5,1.8));
#11613=CARTESIAN_POINT('',(2.925,5.5,0.9));
#11614=CARTESIAN_POINT('Origin',(3.2,5.5,1.8));
#11615=CARTESIAN_POINT('Origin',(-4.,2.9,1.8));
#11616=CARTESIAN_POINT('',(-2.5,3.9,1.8));
#11617=CARTESIAN_POINT('',(-2.5,2.9,1.8));
#11618=CARTESIAN_POINT('',(-2.5,3.9,1.8));
#11619=CARTESIAN_POINT('',(2.5,3.9,1.8));
#11620=CARTESIAN_POINT('',(2.5,3.9,1.8));
#11621=CARTESIAN_POINT('',(2.5,2.9,1.8));
#11622=CARTESIAN_POINT('',(2.5,2.9,1.8));
#11623=CARTESIAN_POINT('',(4.,2.9,1.8));
#11624=CARTESIAN_POINT('',(4.,2.9,1.8));
#11625=CARTESIAN_POINT('',(4.,6.9,1.8));
#11626=CARTESIAN_POINT('',(4.,2.9,1.8));
#11627=CARTESIAN_POINT('',(-4.,6.9,1.8));
#11628=CARTESIAN_POINT('',(4.,6.9,1.8));
#11629=CARTESIAN_POINT('',(-4.,2.9,1.8));
#11630=CARTESIAN_POINT('',(-4.,2.9,1.8));
#11631=CARTESIAN_POINT('',(4.,2.9,1.8));
#11632=CARTESIAN_POINT('Origin',(-4.,2.9,1.));
#11633=CARTESIAN_POINT('',(-4.,2.9,1.));
#11634=CARTESIAN_POINT('',(-4.,2.9,1.8));
#11635=CARTESIAN_POINT('',(-4.,6.9,1.));
#11636=CARTESIAN_POINT('',(-4.,6.9,1.8));
#11637=CARTESIAN_POINT('',(-4.,2.9,1.));
#11638=CARTESIAN_POINT('Origin',(4.,2.9,1.));
#11639=CARTESIAN_POINT('',(4.,2.9,1.));
#11640=CARTESIAN_POINT('',(-4.,2.9,1.));
#11641=CARTESIAN_POINT('',(4.,6.9,1.));
#11642=CARTESIAN_POINT('',(-4.,6.9,1.));
#11643=CARTESIAN_POINT('',(4.,2.9,1.));
#11644=CARTESIAN_POINT('Origin',(4.,2.9,1.8));
#11645=CARTESIAN_POINT('',(4.,2.9,1.));
#11646=CARTESIAN_POINT('',(4.,6.9,1.));
#11647=CARTESIAN_POINT('Origin',(0.,6.9,1.4));
#11648=CARTESIAN_POINT('Origin',(2.5,3.9,1.8));
#11649=CARTESIAN_POINT('',(-2.5,3.9,17.));
#11650=CARTESIAN_POINT('',(-2.5,3.9,1.8));
#11651=CARTESIAN_POINT('',(2.5,3.9,17.));
#11652=CARTESIAN_POINT('',(2.5,3.9,17.));
#11653=CARTESIAN_POINT('',(2.5,3.9,1.8));
#11654=CARTESIAN_POINT('Origin',(2.5,2.9,1.8));
#11655=CARTESIAN_POINT('',(2.5,2.9,17.));
#11656=CARTESIAN_POINT('',(2.5,2.9,17.));
#11657=CARTESIAN_POINT('',(2.5,2.9,1.8));
#11658=CARTESIAN_POINT('Origin',(-2.5,2.9,1.8));
#11659=CARTESIAN_POINT('',(-2.5,2.9,17.));
#11660=CARTESIAN_POINT('',(-2.5,2.9,17.));
#11661=CARTESIAN_POINT('',(-2.5,2.9,1.8));
#11662=CARTESIAN_POINT('Origin',(-2.5,3.9,1.8));
#11663=CARTESIAN_POINT('',(-2.5,3.9,17.));
#11664=CARTESIAN_POINT('Origin',(0.,3.4,17.));
#14404=UNCERTAINTY_MEASURE_WITH_UNIT(LENGTH_MEASURE(0.001),#14513,
'DISTANCE_ACCURACY_VALUE',
'Maximum model space distance between geometric entities at asserted c
onnectivities');
#14455=UNCERTAINTY_MEASURE_WITH_UNIT(LENGTH_MEASURE(0.001),#14513,
'DISTANCE_ACCURACY_VALUE',
'Maximum model space distance between geometric entities at asserted c
onnectivities');
#14461=(
GEOMETRIC_REPRESENTATION_CONTEXT(3)
GLOBAL_UNCERTAINTY_ASSIGNED_CONTEXT((#14404))
GLOBAL_UNIT_ASSIGNED_CONTEXT((#14513,#14515,#14516))
REPRESENTATION_CONTEXT('','3D')
);
#14512=(
GEOMETRIC_REPRESENTATION_CONTEXT(3)
GLOBAL_UNCERTAINTY_ASSIGNED_CONTEXT((#14455))
GLOBAL_UNIT_ASSIGNED_CONTEXT((#14513,#14515,#14516))
REPRESENTATION_CONTEXT('','3D')
);
#14513=(
LENGTH_UNIT()
NAMED_UNIT(*)
SI_UNIT(.CENTI.,.METRE.)
);
#14515=(
NAMED_UNIT(*)
PLANE_ANGLE_UNIT()
SI_UNIT($,.RADIAN.)
);
#14516=(
NAMED_UNIT(*)
SI_UNIT($,.STERADIAN.)
SOLID_ANGLE_UNIT()
);
#14522=SHAPE_DEFINITION_REPRESENTATION(#14578,#14746);
#14578=PRODUCT_DEFINITION_SHAPE('',$,#14803);
#14746=SHAPE_REPRESENTATION('',(#7973),#14461);
#14797=PRODUCT_DEFINITION_CONTEXT('part definition',#14967,'design');
#14803=PRODUCT_DEFINITION('Fixed link','Fixed link',#14859,#14797);
#14859=PRODUCT_DEFINITION_FORMATION('',$,#14974);
#14967=APPLICATION_CONTEXT(
'Core Data for Automotive Mechanical Design Process');
#14968=PRODUCT_CONTEXT('part definition',#14967,'mechanical');
#14974=PRODUCT('Fixed link','Fixed link','Fixed link',(#14968));
#15095=COLOUR_RGB('Off White',0.89,0.88,0.83);
#15096=FILL_AREA_STYLE_COLOUR('',#15095);
#15097=FILL_AREA_STYLE('',(#15096));
#15098=SURFACE_STYLE_FILL_AREA(#15097);
#15099=SURFACE_SIDE_STYLE('',(#15098));
#15100=SURFACE_STYLE_USAGE(.BOTH.,#15099);
#15101=PRESENTATION_STYLE_ASSIGNMENT((#15100));
ENDSEC;
END-ISO-10303-21;
